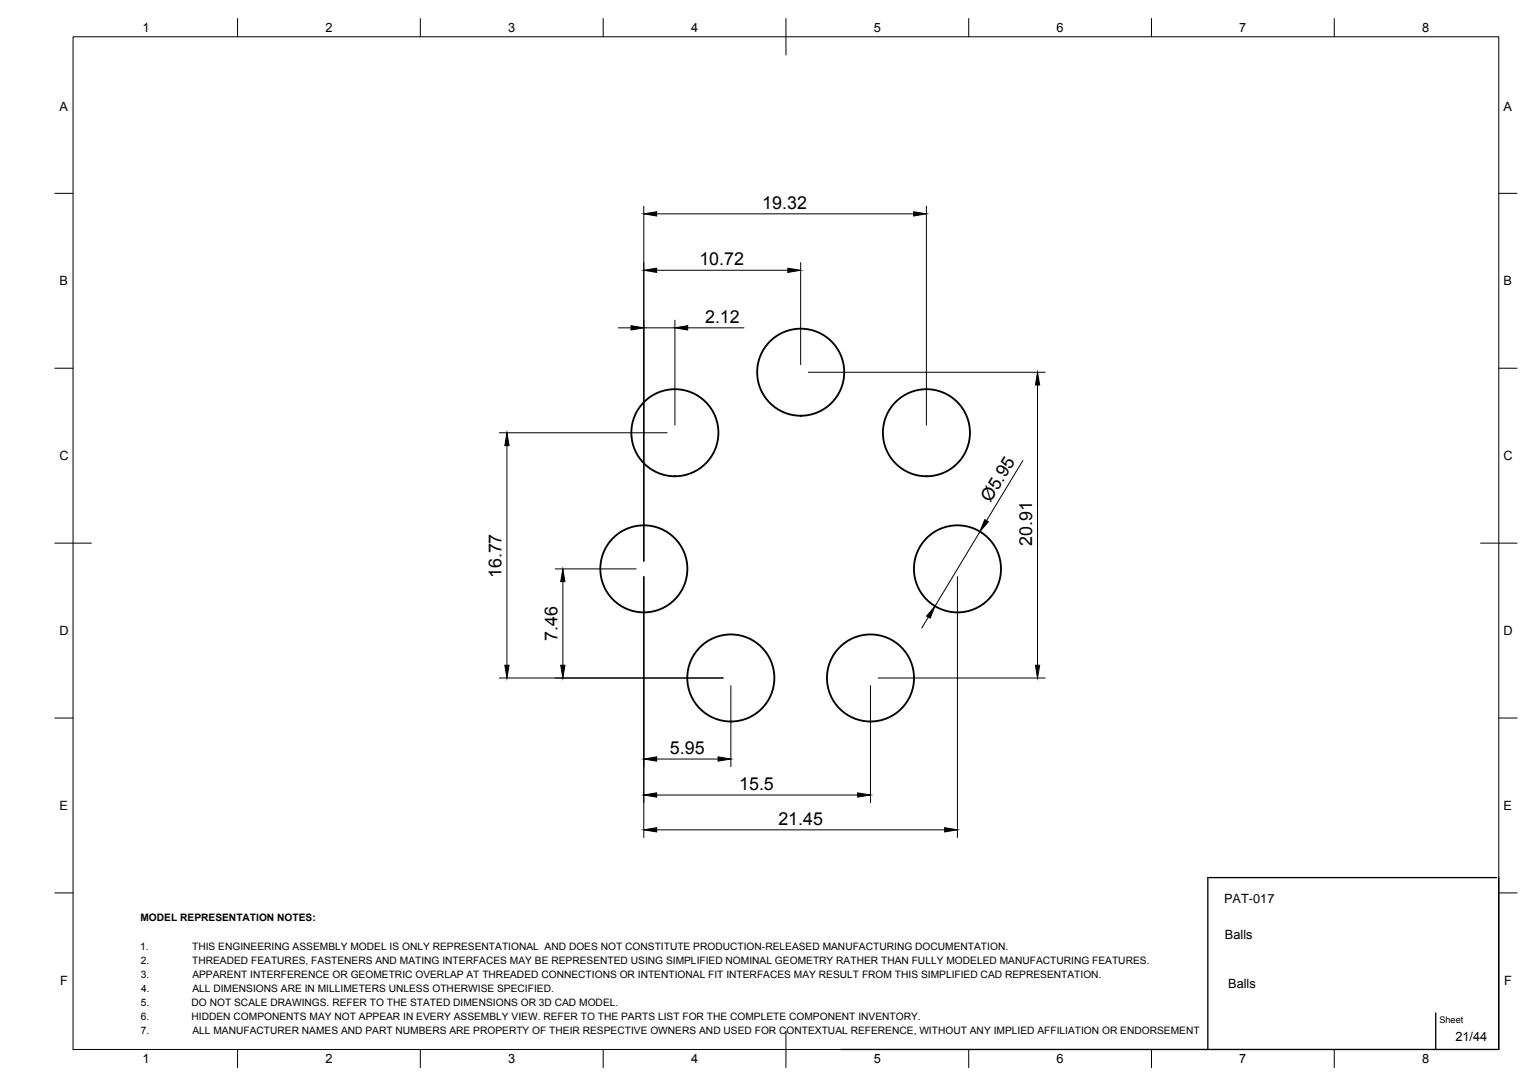
ISO-10303-21;
HEADER;
/* Generated by software containing ST-Developer
 * from STEP Tools, Inc. (www.steptools.com) 
 */

FILE_DESCRIPTION(
/* description */ ('Cam-and-follower valve demonstrator'),
/* implementation_level */ '2;1');

FILE_NAME(
/* name */ 'Balls.step',
/* time_stamp */ '2026-10-28T03:25:17-07:00',
/* author */ (''),
/* organization */ (''),
/* preprocessor_version */ 'ST-DEVELOPER v20.2',
/* originating_system */ 'Autodesk Translation Framework v15.17.0.0',
/* authorisation */ '');

FILE_SCHEMA (('AUTOMOTIVE_DESIGN { 1 0 10303 214 3 1 1 }'));
ENDSEC;

DATA;
#10=MECHANICAL_DESIGN_GEOMETRIC_PRESENTATION_REPRESENTATION('',(#426,#427,#428,#429,#430,#431,#432),#12896);
#293=SPHERICAL_SURFACE('',#6956,0.29765);
#294=SPHERICAL_SURFACE('',#6958,0.29765);
#295=SPHERICAL_SURFACE('',#6960,0.29765);
#296=SPHERICAL_SURFACE('',#6962,0.29765);
#297=SPHERICAL_SURFACE('',#6964,0.29765);
#298=SPHERICAL_SURFACE('',#6966,0.29765);
#299=SPHERICAL_SURFACE('',#6968,0.29765);
#354=SHAPE_REPRESENTATION_RELATIONSHIP('SRR','None',#13071,#390);
#390=ADVANCED_BREP_SHAPE_REPRESENTATION('',(#469,#470,#471,#472,#473,#474,
#475),#12871);
#426=STYLED_ITEM('',(#13330),#469);
#427=STYLED_ITEM('',(#13330),#470);
#428=STYLED_ITEM('',(#13330),#471);
#429=STYLED_ITEM('',(#13330),#472);
#430=STYLED_ITEM('',(#13330),#473);
#431=STYLED_ITEM('',(#13330),#474);
#432=STYLED_ITEM('',(#13330),#475);
#469=MANIFOLD_SOLID_BREP('Body1',#6193);
#470=MANIFOLD_SOLID_BREP('Body2',#6194);
#471=MANIFOLD_SOLID_BREP('Body3',#6195);
#472=MANIFOLD_SOLID_BREP('Body4',#6196);
#473=MANIFOLD_SOLID_BREP('Body5',#6197);
#474=MANIFOLD_SOLID_BREP('Body6',#6198);
#475=MANIFOLD_SOLID_BREP('Body7',#6199);
#813=CIRCLE('',#6957,0.29765);
#814=CIRCLE('',#6959,0.29765);
#815=CIRCLE('',#6961,0.29765);
#816=CIRCLE('',#6963,0.29765);
#817=CIRCLE('',#6965,0.29765);
#818=CIRCLE('',#6967,0.29765);
#819=CIRCLE('',#6969,0.29765);
#1258=FACE_OUTER_BOUND('',#1739,.T.);
#1259=FACE_OUTER_BOUND('',#1740,.T.);
#1260=FACE_OUTER_BOUND('',#1741,.T.);
#1261=FACE_OUTER_BOUND('',#1742,.T.);
#1262=FACE_OUTER_BOUND('',#1743,.T.);
#1263=FACE_OUTER_BOUND('',#1744,.T.);
#1264=FACE_OUTER_BOUND('',#1745,.T.);
#1739=EDGE_LOOP('',(#4819,#4820));
#1740=EDGE_LOOP('',(#4821,#4822));
#1741=EDGE_LOOP('',(#4823,#4824));
#1742=EDGE_LOOP('',(#4825,#4826));
#1743=EDGE_LOOP('',(#4827,#4828));
#1744=EDGE_LOOP('',(#4829,#4830));
#1745=EDGE_LOOP('',(#4831,#4832));
#3079=VERTEX_POINT('',#11566);
#3080=VERTEX_POINT('',#11567);
#3081=VERTEX_POINT('',#11570);
#3082=VERTEX_POINT('',#11571);
#3083=VERTEX_POINT('',#11574);
#3084=VERTEX_POINT('',#11575);
#3085=VERTEX_POINT('',#11578);
#3086=VERTEX_POINT('',#11579);
#3087=VERTEX_POINT('',#11582);
#3088=VERTEX_POINT('',#11583);
#3089=VERTEX_POINT('',#11586);
#3090=VERTEX_POINT('',#11587);
#3091=VERTEX_POINT('',#11590);
#3092=VERTEX_POINT('',#11591);
#3706=EDGE_CURVE('',#3079,#3080,#813,.T.);
#3707=EDGE_CURVE('',#3081,#3082,#814,.T.);
#3708=EDGE_CURVE('',#3083,#3084,#815,.T.);
#3709=EDGE_CURVE('',#3085,#3086,#816,.T.);
#3710=EDGE_CURVE('',#3087,#3088,#817,.T.);
#3711=EDGE_CURVE('',#3089,#3090,#818,.T.);
#3712=EDGE_CURVE('',#3091,#3092,#819,.T.);
#4819=ORIENTED_EDGE('',*,*,#3706,.T.);
#4820=ORIENTED_EDGE('',*,*,#3706,.F.);
#4821=ORIENTED_EDGE('',*,*,#3707,.T.);
#4822=ORIENTED_EDGE('',*,*,#3707,.F.);
#4823=ORIENTED_EDGE('',*,*,#3708,.T.);
#4824=ORIENTED_EDGE('',*,*,#3708,.F.);
#4825=ORIENTED_EDGE('',*,*,#3709,.T.);
#4826=ORIENTED_EDGE('',*,*,#3709,.F.);
#4827=ORIENTED_EDGE('',*,*,#3710,.T.);
#4828=ORIENTED_EDGE('',*,*,#3710,.F.);
#4829=ORIENTED_EDGE('',*,*,#3711,.T.);
#4830=ORIENTED_EDGE('',*,*,#3711,.F.);
#4831=ORIENTED_EDGE('',*,*,#3712,.T.);
#4832=ORIENTED_EDGE('',*,*,#3712,.F.);
#5974=ADVANCED_FACE('',(#1258),#293,.T.);
#5975=ADVANCED_FACE('',(#1259),#294,.T.);
#5976=ADVANCED_FACE('',(#1260),#295,.T.);
#5977=ADVANCED_FACE('',(#1261),#296,.T.);
#5978=ADVANCED_FACE('',(#1262),#297,.T.);
#5979=ADVANCED_FACE('',(#1263),#298,.T.);
#5980=ADVANCED_FACE('',(#1264),#299,.T.);
#6193=CLOSED_SHELL('',(#5974));
#6194=CLOSED_SHELL('',(#5975));
#6195=CLOSED_SHELL('',(#5976));
#6196=CLOSED_SHELL('',(#5977));
#6197=CLOSED_SHELL('',(#5978));
#6198=CLOSED_SHELL('',(#5979));
#6199=CLOSED_SHELL('',(#5980));
#6955=AXIS2_PLACEMENT_3D('',#11564,#8287,#8288);
#6956=AXIS2_PLACEMENT_3D('',#11565,#8289,#8290);
#6957=AXIS2_PLACEMENT_3D('',#11568,#8291,#8292);
#6958=AXIS2_PLACEMENT_3D('',#11569,#8293,#8294);
#6959=AXIS2_PLACEMENT_3D('',#11572,#8295,#8296);
#6960=AXIS2_PLACEMENT_3D('',#11573,#8297,#8298);
#6961=AXIS2_PLACEMENT_3D('',#11576,#8299,#8300);
#6962=AXIS2_PLACEMENT_3D('',#11577,#8301,#8302);
#6963=AXIS2_PLACEMENT_3D('',#11580,#8303,#8304);
#6964=AXIS2_PLACEMENT_3D('',#11581,#8305,#8306);
#6965=AXIS2_PLACEMENT_3D('',#11584,#8307,#8308);
#6966=AXIS2_PLACEMENT_3D('',#11585,#8309,#8310);
#6967=AXIS2_PLACEMENT_3D('',#11588,#8311,#8312);
#6968=AXIS2_PLACEMENT_3D('',#11589,#8313,#8314);
#6969=AXIS2_PLACEMENT_3D('',#11592,#8315,#8316);
#8287=DIRECTION('axis',(0.,0.,1.));
#8288=DIRECTION('refdir',(1.,0.,0.));
#8289=DIRECTION('center_axis',(0.,0.,1.));
#8290=DIRECTION('ref_axis',(1.,0.,0.));
#8291=DIRECTION('center_axis',(1.22464679914735E-16,-1.,0.));
#8292=DIRECTION('ref_axis',(-1.,-1.22464679914735E-16,0.));
#8293=DIRECTION('center_axis',(0.78183148246803,0.,0.623489801858733));
#8294=DIRECTION('ref_axis',(0.623489801858734,0.,-0.78183148246803));
#8295=DIRECTION('center_axis',(7.63554790147315E-17,-1.,-9.57467422477103E-17));
#8296=DIRECTION('ref_axis',(-0.623489801858734,-1.22464679914735E-16,0.78183148246803));
#8297=DIRECTION('center_axis',(0.974927912181824,0.,-0.222520933956314));
#8298=DIRECTION('ref_axis',(-0.222520933956314,0.,-0.974927912181824));
#8299=DIRECTION('center_axis',(-2.7250954951288E-17,-1.,-1.19394234705288E-16));
#8300=DIRECTION('ref_axis',(0.222520933956314,-1.22464679914735E-16,0.974927912181824));
#8301=DIRECTION('center_axis',(0.433883739117558,0.,-0.900968867902419));
#8302=DIRECTION('ref_axis',(-0.900968867902419,0.,-0.433883739117558));
#8303=DIRECTION('center_axis',(-1.10336864020811E-16,-1.,-5.31354332312403E-17));
#8304=DIRECTION('ref_axis',(0.900968867902419,-1.22464679914735E-16,0.433883739117558));
#8305=DIRECTION('center_axis',(-0.433883739117558,0.,-0.900968867902419));
#8306=DIRECTION('ref_axis',(-0.900968867902419,0.,0.433883739117558));
#8307=DIRECTION('center_axis',(-1.10336864020811E-16,-1.,5.31354332312403E-17));
#8308=DIRECTION('ref_axis',(0.900968867902419,-1.22464679914735E-16,-0.433883739117558));
#8309=DIRECTION('center_axis',(-0.974927912181824,0.,-0.222520933956314));
#8310=DIRECTION('ref_axis',(-0.222520933956315,0.,0.974927912181824));
#8311=DIRECTION('center_axis',(-2.7250954951288E-17,-1.,1.19394234705288E-16));
#8312=DIRECTION('ref_axis',(0.222520933956315,-1.22464679914735E-16,-0.974927912181824));
#8313=DIRECTION('center_axis',(-0.78183148246803,0.,0.623489801858734));
#8314=DIRECTION('ref_axis',(0.623489801858733,0.,0.78183148246803));
#8315=DIRECTION('center_axis',(7.63554790147315E-17,-1.,9.57467422477103E-17));
#8316=DIRECTION('ref_axis',(-0.623489801858733,-1.22464679914735E-16,-0.78183148246803));
#11564=CARTESIAN_POINT('',(0.,0.,0.));
#11565=CARTESIAN_POINT('Origin',(1.1,0.,0.));
#11566=CARTESIAN_POINT('',(1.1,-2.23201749654651E-33,0.29765));
#11567=CARTESIAN_POINT('',(1.1,-2.23201749654651E-33,-0.29765));
#11568=CARTESIAN_POINT('Origin',(1.1,0.,0.));
#11569=CARTESIAN_POINT('Origin',(0.685838782044607,0.,-0.860014630714833));
#11570=CARTESIAN_POINT('',(0.918550922801216,-5.31350540756609E-33,-0.674432891191581));
#11571=CARTESIAN_POINT('',(0.453126641287998,8.49470414473068E-34,-1.04559637023808));
#11572=CARTESIAN_POINT('Origin',(0.685838782044607,0.,-0.860014630714833));
#11573=CARTESIAN_POINT('Origin',(-0.244773027351946,0.,-1.07242070340001));
#11574=CARTESIAN_POINT('',(0.0454142657089739,-2.23201749654651E-33,-1.1386540593921));
#11575=CARTESIAN_POINT('',(-0.534960320412865,-2.23201749654651E-33,-1.00618734740791));
#11576=CARTESIAN_POINT('Origin',(-0.244773027351946,0.,-1.07242070340001));
#11577=CARTESIAN_POINT('Origin',(-0.991065754692661,0.,-0.477272113029314));
#11578=CARTESIAN_POINT('',(-0.86192025974432,8.49470414473067E-34,-0.745445496560469));
#11579=CARTESIAN_POINT('',(-1.120211249641,-5.31350540756609E-33,-0.209098729498159));
#11580=CARTESIAN_POINT('Origin',(-0.991065754692661,0.,-0.477272113029314));
#11581=CARTESIAN_POINT('Origin',(-0.991065754692661,0.,0.477272113029314));
#11582=CARTESIAN_POINT('',(-1.120211249641,-2.23201749654651E-33,0.209098729498159));
#11583=CARTESIAN_POINT('',(-0.86192025974432,-2.23201749654651E-33,0.745445496560469));
#11584=CARTESIAN_POINT('Origin',(-0.991065754692661,0.,0.477272113029314));
#11585=CARTESIAN_POINT('Origin',(-0.244773027351946,0.,1.07242070340001));
#11586=CARTESIAN_POINT('',(-0.534960320412866,-2.23201749654651E-33,1.00618734740791));
#11587=CARTESIAN_POINT('',(0.0454142657089737,-2.23201749654651E-33,1.1386540593921));
#11588=CARTESIAN_POINT('Origin',(-0.244773027351946,0.,1.07242070340001));
#11589=CARTESIAN_POINT('Origin',(0.685838782044607,0.,0.860014630714833));
#11590=CARTESIAN_POINT('',(0.453126641287998,-2.23201749654651E-33,1.04559637023808));
#11591=CARTESIAN_POINT('',(0.918550922801216,-2.23201749654651E-33,0.674432891191581));
#11592=CARTESIAN_POINT('Origin',(0.685838782044607,0.,0.860014630714833));
#12828=UNCERTAINTY_MEASURE_WITH_UNIT(LENGTH_MEASURE(0.001),#12897,
'DISTANCE_ACCURACY_VALUE',
'Maximum model space distance between geometric entities at asserted c
onnectivities');
#12853=UNCERTAINTY_MEASURE_WITH_UNIT(LENGTH_MEASURE(0.001),#12897,
'DISTANCE_ACCURACY_VALUE',
'Maximum model space distance between geometric entities at asserted c
onnectivities');
#12871=(
GEOMETRIC_REPRESENTATION_CONTEXT(3)
GLOBAL_UNCERTAINTY_ASSIGNED_CONTEXT((#12828))
GLOBAL_UNIT_ASSIGNED_CONTEXT((#12897,#12899,#12900))
REPRESENTATION_CONTEXT('','3D')
);
#12896=(
GEOMETRIC_REPRESENTATION_CONTEXT(3)
GLOBAL_UNCERTAINTY_ASSIGNED_CONTEXT((#12853))
GLOBAL_UNIT_ASSIGNED_CONTEXT((#12897,#12899,#12900))
REPRESENTATION_CONTEXT('','3D')
);
#12897=(
LENGTH_UNIT()
NAMED_UNIT(*)
SI_UNIT(.CENTI.,.METRE.)
);
#12899=(
NAMED_UNIT(*)
PLANE_ANGLE_UNIT()
SI_UNIT($,.RADIAN.)
);
#12900=(
NAMED_UNIT(*)
SI_UNIT($,.STERADIAN.)
SOLID_ANGLE_UNIT()
);
#12918=SHAPE_DEFINITION_REPRESENTATION(#12960,#13071);
#12960=PRODUCT_DEFINITION_SHAPE('',$,#13114);
#13071=SHAPE_REPRESENTATION('',(#6955),#12871);
#13096=PRODUCT_DEFINITION_CONTEXT('part definition',#13224,'design');
#13114=PRODUCT_DEFINITION('Balls','Balls',#13156,#13096);
#13156=PRODUCT_DEFINITION_FORMATION('',$,#13243);
#13224=APPLICATION_CONTEXT(
'Core Data for Automotive Mechanical Design Process');
#13225=PRODUCT_CONTEXT('part definition',#13224,'mechanical');
#13243=PRODUCT('Balls','Balls','Balls',(#13225));
#13324=COLOUR_RGB('Grey',0.48,0.52,0.57);
#13325=FILL_AREA_STYLE_COLOUR('',#13324);
#13326=FILL_AREA_STYLE('',(#13325));
#13327=SURFACE_STYLE_FILL_AREA(#13326);
#13328=SURFACE_SIDE_STYLE('',(#13327));
#13329=SURFACE_STYLE_USAGE(.BOTH.,#13328);
#13330=PRESENTATION_STYLE_ASSIGNMENT((#13329));
ENDSEC;
END-ISO-10303-21;
